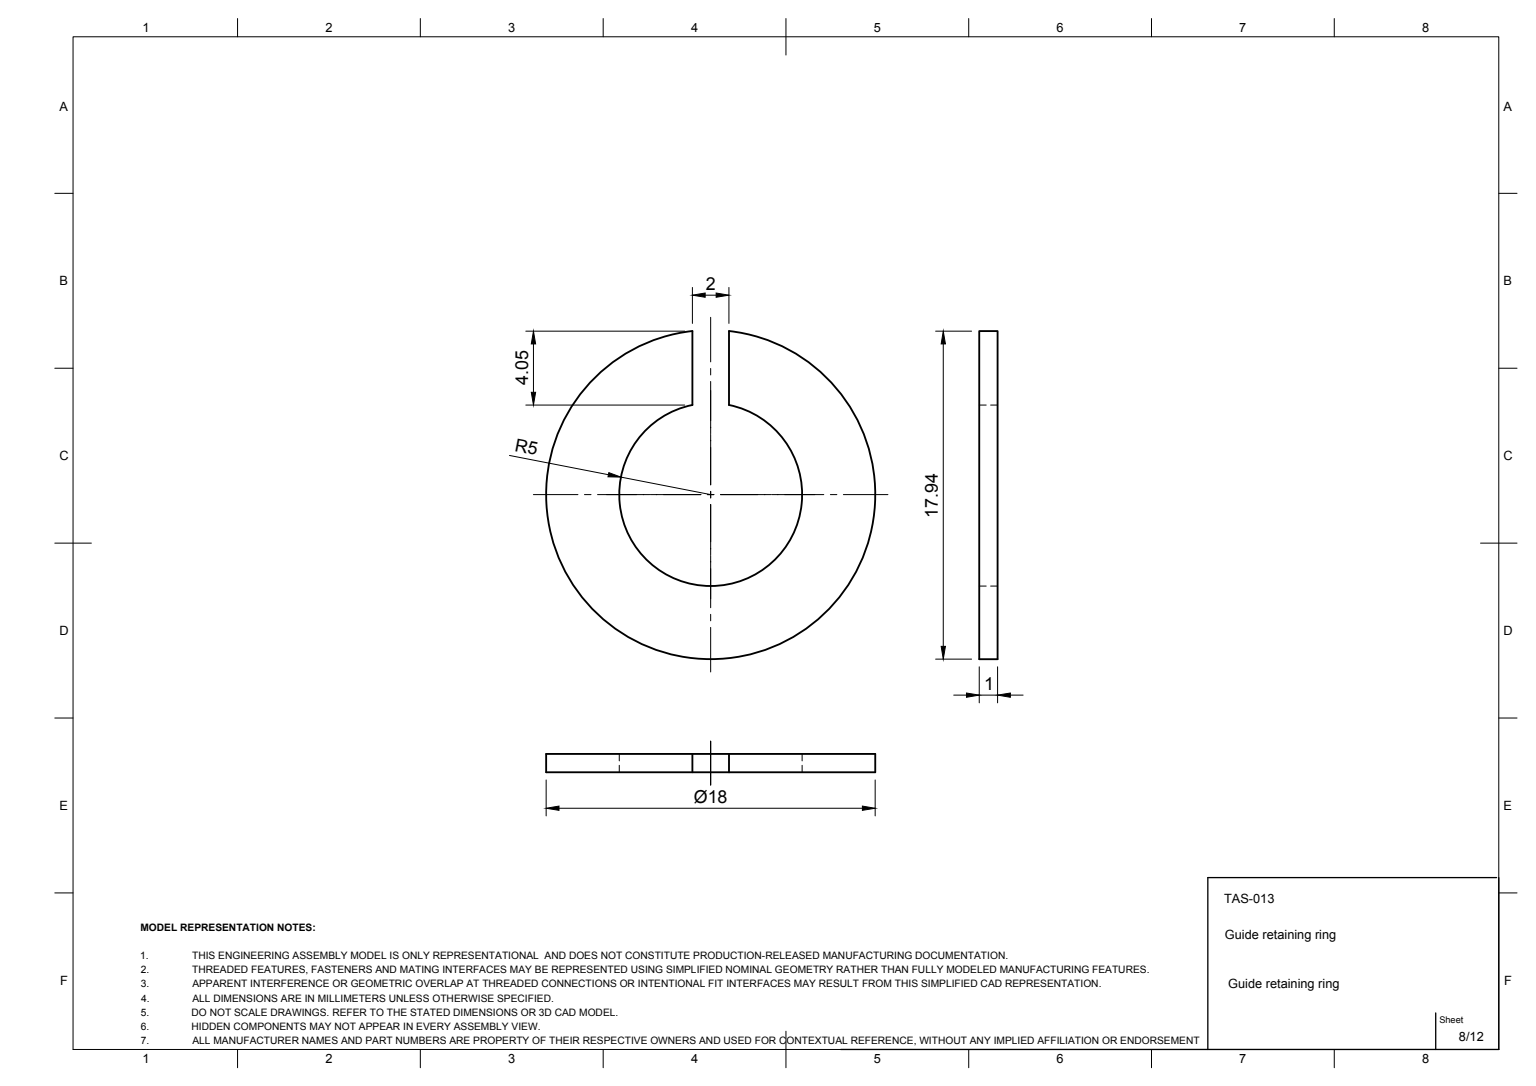
ISO-10303-21;
HEADER;
/* Generated by software containing ST-Developer
 * from STEP Tools, Inc. (www.steptools.com) 
 */

FILE_DESCRIPTION(
/* description */ (
'Independent guided parallel-jaw bracket clamp. Two12mm guide rods, re
placeable bronze sleeves, captured swiveling spindle, replaceable jaw 
pads and modeled M16x2 screw. Native slider/revolute joints linked2mm 
per revolution. Nominal opening0..122 with initial28mm. Base and two i
dentical supports welded. Standard fits, weld details and clamp load r
equire engineering selection.'),
/* implementation_level */ '2;1');

FILE_NAME(
/* name */ 'Guide retaining ring.step',
/* time_stamp */ '2026-11-14T09:15:44-08:00',
/* author */ (''),
/* organization */ (''),
/* preprocessor_version */ 'ST-DEVELOPER v20.2',
/* originating_system */ 'Autodesk Translation Framework v15.17.0.0',
/* authorisation */ '');

FILE_SCHEMA (('AUTOMOTIVE_DESIGN { 1 0 10303 214 3 1 1 }'));
ENDSEC;

DATA;
#10=MECHANICAL_DESIGN_GEOMETRIC_PRESENTATION_REPRESENTATION('',(#923),#105806);
#899=SHAPE_REPRESENTATION_RELATIONSHIP('SRR','None',#105867,#911);
#911=ADVANCED_BREP_SHAPE_REPRESENTATION('',(#935),#105802);
#923=STYLED_ITEM('',(#105932),#935);
#935=MANIFOLD_SOLID_BREP('Body1',#7210);
#1047=PLANE('',#7648);
#1048=PLANE('',#7649);
#1049=PLANE('',#7650);
#1050=PLANE('',#7657);
#1283=FACE_OUTER_BOUND('',#1608,.T.);
#1284=FACE_OUTER_BOUND('',#1609,.T.);
#1285=FACE_OUTER_BOUND('',#1610,.T.);
#1286=FACE_OUTER_BOUND('',#1611,.T.);
#1287=FACE_OUTER_BOUND('',#1612,.T.);
#1288=FACE_OUTER_BOUND('',#1613,.T.);
#1608=EDGE_LOOP('',(#6317,#6318,#6319,#6320));
#1609=EDGE_LOOP('',(#6321,#6322,#6323,#6324));
#1610=EDGE_LOOP('',(#6325,#6326,#6327,#6328));
#1611=EDGE_LOOP('',(#6329,#6330,#6331,#6332));
#1612=EDGE_LOOP('',(#6333,#6334,#6335,#6336));
#1613=EDGE_LOOP('',(#6337,#6338,#6339,#6340));
#1892=LINE('',#88799,#2172);
#1893=LINE('',#88801,#2173);
#1894=LINE('',#88803,#2174);
#1895=LINE('',#88804,#2175);
#1896=LINE('',#88808,#2176);
#1897=LINE('',#88810,#2177);
#1898=LINE('',#88812,#2178);
#1899=LINE('',#88813,#2179);
#2172=VECTOR('',#8571,10.);
#2173=VECTOR('',#8572,10.);
#2174=VECTOR('',#8573,10.);
#2175=VECTOR('',#8574,10.);
#2176=VECTOR('',#8577,10.);
#2177=VECTOR('',#8578,10.);
#2178=VECTOR('',#8579,10.);
#2179=VECTOR('',#8580,10.);
#2307=CIRCLE('',#7651,9.);
#2308=CIRCLE('',#7652,5.);
#2309=CIRCLE('',#7654,5.);
#2310=CIRCLE('',#7656,9.);
#3085=VERTEX_POINT('',#88797);
#3086=VERTEX_POINT('',#88798);
#3087=VERTEX_POINT('',#88800);
#3088=VERTEX_POINT('',#88802);
#3089=VERTEX_POINT('',#88806);
#3090=VERTEX_POINT('',#88807);
#3091=VERTEX_POINT('',#88809);
#3092=VERTEX_POINT('',#88811);
#4203=EDGE_CURVE('',#3085,#3086,#1892,.T.);
#4204=EDGE_CURVE('',#3087,#3085,#1893,.T.);
#4205=EDGE_CURVE('',#3088,#3087,#1894,.T.);
#4206=EDGE_CURVE('',#3086,#3088,#1895,.T.);
#4207=EDGE_CURVE('',#3089,#3090,#1896,.T.);
#4208=EDGE_CURVE('',#3091,#3089,#1897,.T.);
#4209=EDGE_CURVE('',#3092,#3091,#1898,.T.);
#4210=EDGE_CURVE('',#3090,#3092,#1899,.T.);
#4211=EDGE_CURVE('',#3087,#3092,#2307,.T.);
#4212=EDGE_CURVE('',#3090,#3085,#2308,.T.);
#4213=EDGE_CURVE('',#3089,#3086,#2309,.T.);
#4214=EDGE_CURVE('',#3088,#3091,#2310,.T.);
#6317=ORIENTED_EDGE('',*,*,#4203,.F.);
#6318=ORIENTED_EDGE('',*,*,#4204,.F.);
#6319=ORIENTED_EDGE('',*,*,#4205,.F.);
#6320=ORIENTED_EDGE('',*,*,#4206,.F.);
#6321=ORIENTED_EDGE('',*,*,#4207,.F.);
#6322=ORIENTED_EDGE('',*,*,#4208,.F.);
#6323=ORIENTED_EDGE('',*,*,#4209,.F.);
#6324=ORIENTED_EDGE('',*,*,#4210,.F.);
#6325=ORIENTED_EDGE('',*,*,#4210,.T.);
#6326=ORIENTED_EDGE('',*,*,#4211,.F.);
#6327=ORIENTED_EDGE('',*,*,#4204,.T.);
#6328=ORIENTED_EDGE('',*,*,#4212,.F.);
#6329=ORIENTED_EDGE('',*,*,#4207,.T.);
#6330=ORIENTED_EDGE('',*,*,#4212,.T.);
#6331=ORIENTED_EDGE('',*,*,#4203,.T.);
#6332=ORIENTED_EDGE('',*,*,#4213,.F.);
#6333=ORIENTED_EDGE('',*,*,#4209,.T.);
#6334=ORIENTED_EDGE('',*,*,#4214,.F.);
#6335=ORIENTED_EDGE('',*,*,#4205,.T.);
#6336=ORIENTED_EDGE('',*,*,#4211,.T.);
#6337=ORIENTED_EDGE('',*,*,#4208,.T.);
#6338=ORIENTED_EDGE('',*,*,#4213,.T.);
#6339=ORIENTED_EDGE('',*,*,#4206,.T.);
#6340=ORIENTED_EDGE('',*,*,#4214,.T.);
#6897=CYLINDRICAL_SURFACE('',#7653,5.);
#6898=CYLINDRICAL_SURFACE('',#7655,9.);
#7148=ADVANCED_FACE('',(#1283),#1047,.F.);
#7149=ADVANCED_FACE('',(#1284),#1048,.F.);
#7150=ADVANCED_FACE('',(#1285),#1049,.F.);
#7151=ADVANCED_FACE('',(#1286),#6897,.F.);
#7152=ADVANCED_FACE('',(#1287),#6898,.T.);
#7153=ADVANCED_FACE('',(#1288),#1050,.T.);
#7210=CLOSED_SHELL('',(#7148,#7149,#7150,#7151,#7152,#7153));
#7647=AXIS2_PLACEMENT_3D('',#88795,#8567,#8568);
#7648=AXIS2_PLACEMENT_3D('',#88796,#8569,#8570);
#7649=AXIS2_PLACEMENT_3D('',#88805,#8575,#8576);
#7650=AXIS2_PLACEMENT_3D('',#88814,#8581,#8582);
#7651=AXIS2_PLACEMENT_3D('',#88815,#8583,#8584);
#7652=AXIS2_PLACEMENT_3D('',#88816,#8585,#8586);
#7653=AXIS2_PLACEMENT_3D('',#88817,#8587,#8588);
#7654=AXIS2_PLACEMENT_3D('',#88818,#8589,#8590);
#7655=AXIS2_PLACEMENT_3D('',#88819,#8591,#8592);
#7656=AXIS2_PLACEMENT_3D('',#88820,#8593,#8594);
#7657=AXIS2_PLACEMENT_3D('',#88821,#8595,#8596);
#8567=DIRECTION('axis',(0.,0.,1.));
#8568=DIRECTION('refdir',(1.,0.,0.));
#8569=DIRECTION('center_axis',(-1.,0.,0.));
#8570=DIRECTION('ref_axis',(0.,1.,0.));
#8571=DIRECTION('',(0.,0.,1.));
#8572=DIRECTION('',(0.,-1.,0.));
#8573=DIRECTION('',(0.,0.,-1.));
#8574=DIRECTION('',(0.,1.,0.));
#8575=DIRECTION('center_axis',(1.,0.,0.));
#8576=DIRECTION('ref_axis',(0.,-1.,0.));
#8577=DIRECTION('',(0.,0.,-1.));
#8578=DIRECTION('',(0.,-1.,0.));
#8579=DIRECTION('',(0.,0.,1.));
#8580=DIRECTION('',(0.,1.,0.));
#8581=DIRECTION('center_axis',(0.,0.,1.));
#8582=DIRECTION('ref_axis',(1.,0.,0.));
#8583=DIRECTION('center_axis',(0.,0.,1.));
#8584=DIRECTION('ref_axis',(1.,0.,0.));
#8585=DIRECTION('center_axis',(0.,0.,-1.));
#8586=DIRECTION('ref_axis',(1.,0.,0.));
#8587=DIRECTION('center_axis',(0.,0.,1.));
#8588=DIRECTION('ref_axis',(6.12323399573677E-17,-1.,0.));
#8589=DIRECTION('center_axis',(0.,0.,-1.));
#8590=DIRECTION('ref_axis',(1.,0.,0.));
#8591=DIRECTION('center_axis',(0.,0.,1.));
#8592=DIRECTION('ref_axis',(6.12323399573677E-17,-1.,0.));
#8593=DIRECTION('center_axis',(0.,0.,1.));
#8594=DIRECTION('ref_axis',(1.,0.,0.));
#8595=DIRECTION('center_axis',(0.,0.,1.));
#8596=DIRECTION('ref_axis',(1.,0.,0.));
#88795=CARTESIAN_POINT('',(0.,0.,0.));
#88796=CARTESIAN_POINT('Origin',(-1.,0.,1.));
#88797=CARTESIAN_POINT('',(-1.,4.89897948556636,0.));
#88798=CARTESIAN_POINT('',(-1.,4.89897948556636,1.));
#88799=CARTESIAN_POINT('',(-1.,4.89897948556636,0.));
#88800=CARTESIAN_POINT('',(-1.,8.94427190999916,0.));
#88801=CARTESIAN_POINT('',(-1.,0.,0.));
#88802=CARTESIAN_POINT('',(-1.,8.94427190999916,1.));
#88803=CARTESIAN_POINT('',(-1.,8.94427190999916,0.));
#88804=CARTESIAN_POINT('',(-1.,0.,1.));
#88805=CARTESIAN_POINT('Origin',(1.,18.,1.));
#88806=CARTESIAN_POINT('',(1.,4.89897948556636,1.));
#88807=CARTESIAN_POINT('',(1.,4.89897948556636,0.));
#88808=CARTESIAN_POINT('',(1.,4.89897948556636,0.));
#88809=CARTESIAN_POINT('',(1.,8.94427190999916,1.));
#88810=CARTESIAN_POINT('',(1.,9.,1.));
#88811=CARTESIAN_POINT('',(1.,8.94427190999916,0.));
#88812=CARTESIAN_POINT('',(1.,8.94427190999916,0.));
#88813=CARTESIAN_POINT('',(1.,9.,0.));
#88814=CARTESIAN_POINT('Origin',(0.,0.,0.));
#88815=CARTESIAN_POINT('Origin',(0.,0.,0.));
#88816=CARTESIAN_POINT('Origin',(0.,0.,0.));
#88817=CARTESIAN_POINT('Origin',(0.,0.,0.));
#88818=CARTESIAN_POINT('Origin',(0.,0.,1.));
#88819=CARTESIAN_POINT('Origin',(0.,0.,0.));
#88820=CARTESIAN_POINT('Origin',(0.,0.,1.));
#88821=CARTESIAN_POINT('Origin',(0.,0.,1.));
#105788=UNCERTAINTY_MEASURE_WITH_UNIT(LENGTH_MEASURE(0.01),#105807,
'DISTANCE_ACCURACY_VALUE',
'Maximum model space distance between geometric entities at asserted c
onnectivities');
#105792=UNCERTAINTY_MEASURE_WITH_UNIT(LENGTH_MEASURE(0.01),#105807,
'DISTANCE_ACCURACY_VALUE',
'Maximum model space distance between geometric entities at asserted c
onnectivities');
#105802=(
GEOMETRIC_REPRESENTATION_CONTEXT(3)
GLOBAL_UNCERTAINTY_ASSIGNED_CONTEXT((#105788))
GLOBAL_UNIT_ASSIGNED_CONTEXT((#105807,#105809,#105810))
REPRESENTATION_CONTEXT('','3D')
);
#105806=(
GEOMETRIC_REPRESENTATION_CONTEXT(3)
GLOBAL_UNCERTAINTY_ASSIGNED_CONTEXT((#105792))
GLOBAL_UNIT_ASSIGNED_CONTEXT((#105807,#105809,#105810))
REPRESENTATION_CONTEXT('','3D')
);
#105807=(
LENGTH_UNIT()
NAMED_UNIT(*)
SI_UNIT(.MILLI.,.METRE.)
);
#105809=(
NAMED_UNIT(*)
PLANE_ANGLE_UNIT()
SI_UNIT($,.RADIAN.)
);
#105810=(
NAMED_UNIT(*)
SI_UNIT($,.STERADIAN.)
SOLID_ANGLE_UNIT()
);
#105820=SHAPE_DEFINITION_REPRESENTATION(#105833,#105867);
#105833=PRODUCT_DEFINITION_SHAPE('',$,#105881);
#105867=SHAPE_REPRESENTATION('',(#7647),#105802);
#105871=PRODUCT_DEFINITION_CONTEXT('part definition',#105912,'design');
#105881=PRODUCT_DEFINITION('Guide retaining ring',
'Guide retaining ring',#105894,#105871);
#105894=PRODUCT_DEFINITION_FORMATION('',$,#105923);
#105912=APPLICATION_CONTEXT(
'Core Data for Automotive Mechanical Design Process');
#105913=PRODUCT_CONTEXT('part definition',#105912,'mechanical');
#105923=PRODUCT('Guide retaining ring','Guide retaining ring',$,(#105913));
#105932=PRESENTATION_STYLE_ASSIGNMENT((#105938));
#105938=SURFACE_STYLE_USAGE(.BOTH.,#105944);
#105944=SURFACE_SIDE_STYLE('',(#105950));
#105950=SURFACE_STYLE_FILL_AREA(#105956);
#105956=FILL_AREA_STYLE('Opaque(64,72,82)',(#105962));
#105962=FILL_AREA_STYLE_COLOUR('Opaque(64,72,82)',#105968);
#105968=COLOUR_RGB('Opaque(64,72,82)',0.250980392156863,0.282352941176471,
0.32156862745098);
ENDSEC;
END-ISO-10303-21;
